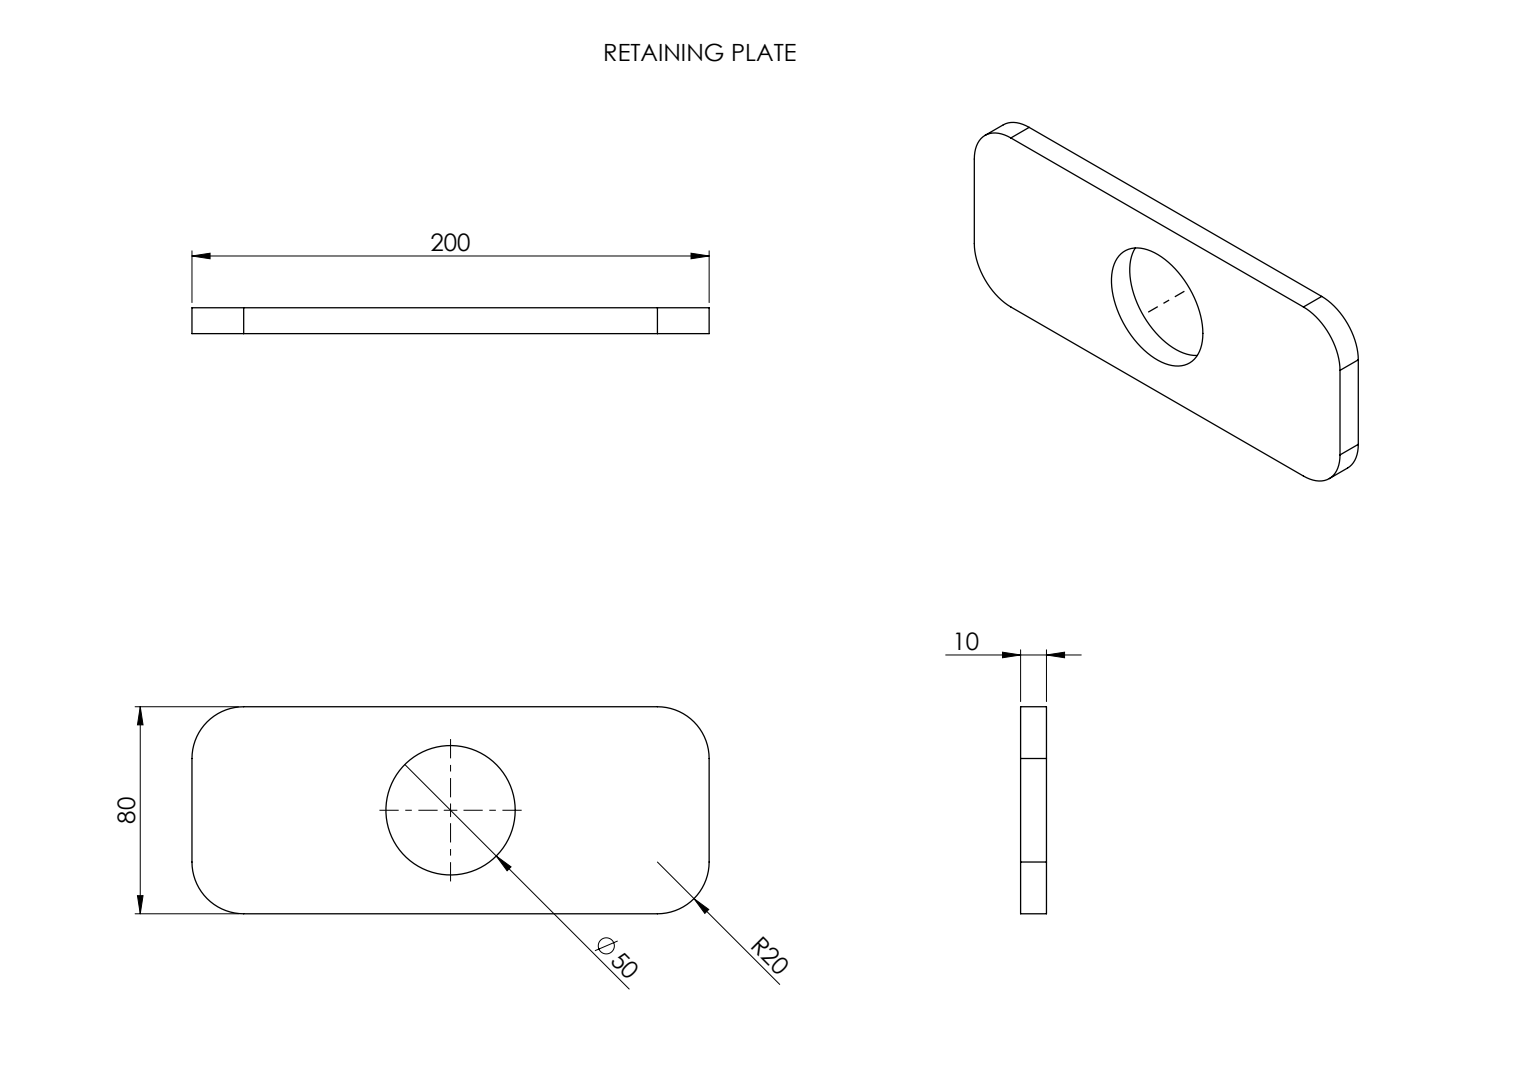
ISO-10303-21;
HEADER;
FILE_DESCRIPTION (('STEP AP203'),
    '1' );
FILE_NAME ('retaining plate.step',
    '2026-09-28T05:57:06',
    ( '' ),
    ( '' ),
    'SwSTEP 2.0',
    'SolidWorks 2026',
    '' );
FILE_SCHEMA (( 'AUTOMOTIVE_DESIGN' ));
ENDSEC;

DATA;
#122=DIRECTION ( 'NONE',  ( -1.000000000000000000, 0.000000000000000000, 0.000000000000000000 ) ) ;
#133=AXIS2_PLACEMENT_3D ( 'NONE', #27318, #14555, #30777 ) ;
#134=VERTEX_POINT ( 'NONE', #10468 ) ;
#200=CYLINDRICAL_SURFACE ( 'NONE', #38257, 25.00000000000000000 ) ;
#235=CARTESIAN_POINT ( 'NONE',  ( 0.000000000000000000, 0.000000000000000000, -170.0000000000000000 ) ) ;
#587=VERTEX_POINT ( 'NONE', #37224 ) ;
#645=EDGE_CURVE ( 'NONE', #15029, #36871, #9699, .T. ) ;
#867=CARTESIAN_POINT ( 'NONE',  ( 80.00000000000002842, 19.99999999999999289, -160.0000000000000000 ) ) ;
#917=DIRECTION ( 'NONE',  ( 0.000000000000000000, 0.000000000000000000, -1.000000000000000000 ) ) ;
#1054=VERTEX_POINT ( 'NONE', #16453 ) ;
#1121=CIRCLE ( 'NONE', #7312, 20.00000000000000355 ) ;
#1204=MANIFOLD_SOLID_BREP ( 'Fillet1', #25326 ) ;
#1238=VECTOR ( 'NONE', #42446, 1000.000000000000000 ) ;
#1422=DIRECTION ( 'NONE',  ( -0.000000000000000000, -0.000000000000000000, 1.000000000000000000 ) ) ;
#1650=VERTEX_POINT ( 'NONE', #15142 ) ;
#1704=ORIENTED_EDGE ( 'NONE', *, *, #24624, .F. ) ;
#1835=EDGE_CURVE ( 'NONE', #1650, #37987, #25230, .T. ) ;
#2068=EDGE_LOOP ( 'NONE', ( #40227, #42312 ) ) ;
#2131=ORIENTED_EDGE ( 'NONE', *, *, #9361, .F. ) ;
#2180=LINE ( 'NONE', #18985, #13807 ) ;
#2200=VECTOR ( 'NONE', #3034, 1000.000000000000000 ) ;
#2225=FACE_OUTER_BOUND ( 'NONE', #37868, .T. ) ;
#2336=DIRECTION ( 'NONE',  ( -1.000000000000000000, 0.000000000000000000, 0.000000000000000000 ) ) ;
#2490=AXIS2_PLACEMENT_3D ( 'NONE', #26366, #42534, #23345 ) ;
#2545=DIRECTION ( 'NONE',  ( 0.000000000000000000, 0.000000000000000000, -1.000000000000000000 ) ) ;
#2726=AXIS2_PLACEMENT_3D ( 'NONE', #867, #39910, #20909 ) ;
#2917=DIRECTION ( 'NONE',  ( 0.000000000000000000, 0.000000000000000000, -1.000000000000000000 ) ) ;
#3034=DIRECTION ( 'NONE',  ( -0.000000000000000000, -0.000000000000000000, 1.000000000000000000 ) ) ;
#3160=DIRECTION ( 'NONE',  ( -0.000000000000000000, -0.000000000000000000, -1.000000000000000000 ) ) ;
#3228=VERTEX_POINT ( 'NONE', #30090 ) ;
#3281=PRODUCT_DEFINITION ( 'UNKNOWN', '', #22864, #26130 ) ;
#3291=AXIS2_PLACEMENT_3D ( 'NONE', #10282, #23469, #36616 ) ;
#3398=VECTOR ( 'NONE', #23149, 1000.000000000000000 ) ;
#3399=FACE_BOUND ( 'NONE', #39258, .T. ) ;
#3599=DIRECTION ( 'NONE',  ( -1.000000000000000000, 0.000000000000000000, 0.000000000000000000 ) ) ;
#3726=DIRECTION ( 'NONE',  ( -1.000000000000000000, -1.734723475976806848E-16, 0.000000000000000000 ) ) ;
#3807=CIRCLE ( 'NONE', #15519, 20.00000000000000355 ) ;
#3812=ORIENTED_EDGE ( 'NONE', *, *, #16436, .F. ) ;
#3857=ORIENTED_EDGE ( 'NONE', *, *, #28973, .F. ) ;
#3901=VECTOR ( 'NONE', #38849, 1000.000000000000000 ) ;
#4172=VERTEX_POINT ( 'NONE', #30883 ) ;
#4780=CARTESIAN_POINT ( 'NONE',  ( -99.99999999999994316, 19.99999999999998934, -160.0000000000000000 ) ) ;
#4830=DIRECTION ( 'NONE',  ( 0.000000000000000000, 0.000000000000000000, -1.000000000000000000 ) ) ;
#4866=DIRECTION ( 'NONE',  ( 0.000000000000000000, 0.000000000000000000, -1.000000000000000000 ) ) ;
#4920=DIRECTION ( 'NONE',  ( 0.000000000000000000, 0.000000000000000000, -1.000000000000000000 ) ) ;
#5144=ORIENTED_EDGE ( 'NONE', *, *, #23603, .F. ) ;
#5298=( NAMED_UNIT ( * ) SI_UNIT ( $, .STERADIAN. ) SOLID_ANGLE_UNIT ( ) );
#5409=CARTESIAN_POINT ( 'NONE',  ( -99.99999999999994316, 39.99999999999999289, -160.0000000000000000 ) ) ;
#5497=ORIENTED_EDGE ( 'NONE', *, *, #20467, .F. ) ;
#5582=AXIS2_PLACEMENT_3D ( 'NONE', #18873, #12589, #31631 ) ;
#5609=EDGE_LOOP ( 'NONE', ( #14936, #24531, #13344, #38796 ) ) ;
#5623=EDGE_LOOP ( 'NONE', ( #1704, #31810, #14532, #33862 ) ) ;
#6178=VECTOR ( 'NONE', #4830, 1000.000000000000000 ) ;
#6245=ORIENTED_EDGE ( 'NONE', *, *, #24624, .T. ) ;
#6332=VECTOR ( 'NONE', #39526, 1000.000000000000000 ) ;
#6411=CARTESIAN_POINT ( 'NONE',  ( 100.0000000000000284, -40.00000000000001421, -160.0000000000000000 ) ) ;
#6686=LINE ( 'NONE', #36256, #2200 ) ;
#6890=ORIENTED_EDGE ( 'NONE', *, *, #8772, .T. ) ;
#6921=ORIENTED_EDGE ( 'NONE', *, *, #32093, .F. ) ;
#6955=FACE_OUTER_BOUND ( 'NONE', #37730, .T. ) ;
#7119=DIRECTION ( 'NONE',  ( -0.000000000000000000, -0.000000000000000000, -1.000000000000000000 ) ) ;
#7120=DIRECTION ( 'NONE',  ( -0.000000000000000000, -0.000000000000000000, 1.000000000000000000 ) ) ;
#7230=ADVANCED_FACE ( 'NONE', ( #39848 ), #16746, .F. ) ;
#7298=DIRECTION ( 'NONE',  ( 0.000000000000000000, 0.000000000000000000, 1.000000000000000000 ) ) ;
#7312=AXIS2_PLACEMENT_3D ( 'NONE', #35263, #14357, #27554 ) ;
#7469=ADVANCED_FACE ( 'NONE', ( #32970, #3399 ), #16534, .F. ) ;
#7703=APPLICATION_CONTEXT ( 'configuration controlled 3d designs of mechanical parts and assemblies' ) ;
#7767=CARTESIAN_POINT ( 'NONE',  ( -79.99999999999994316, -20.00000000000000711, -160.0000000000000000 ) ) ;
#7802=FACE_OUTER_BOUND ( 'NONE', #41194, .T. ) ;
#7902=DIRECTION ( 'NONE',  ( 0.000000000000000000, 0.000000000000000000, 1.000000000000000000 ) ) ;
#8162=CARTESIAN_POINT ( 'NONE',  ( 0.000000000000000000, 0.000000000000000000, -170.0000000000000000 ) ) ;
#8437=EDGE_CURVE ( 'NONE', #3228, #21146, #34411, .T. ) ;
#8559=LINE ( 'NONE', #24974, #41909 ) ;
#8607=DIRECTION ( 'NONE',  ( 1.000000000000000000, -3.469446951953614805E-17, 0.000000000000000000 ) ) ;
#8772=EDGE_CURVE ( 'NONE', #21146, #4172, #25761, .T. ) ;
#8901=EDGE_CURVE ( 'NONE', #1054, #27758, #21322, .T. ) ;
#8918=CIRCLE ( 'NONE', #16462, 25.00000000000000000 ) ;
#9272=MECHANICAL_CONTEXT ( 'NONE', #7703, 'mechanical' ) ;
#9361=EDGE_CURVE ( 'NONE', #36871, #15029, #8918, .T. ) ;
#9371=ORIENTED_EDGE ( 'NONE', *, *, #8772, .F. ) ;
#9378=SHAPE_REPRESENTATION_RELATIONSHIP ( 'NONE' , 'NONE' ,  #10057, #19190 ) ;
#9407=VERTEX_POINT ( 'NONE', #26337 ) ;
#9447=LINE ( 'NONE', #31923, #1238 ) ;
#9492=ORIENTED_EDGE ( 'NONE', *, *, #21192, .T. ) ;
#9586=EDGE_LOOP ( 'NONE', ( #5144, #34825, #5497, #32629 ) ) ;
#9592=ADVANCED_FACE ( 'NONE', ( #26124 ), #22894, .T. ) ;
#9637=CYLINDRICAL_SURFACE ( 'NONE', #9748, 20.00000000000000355 ) ;
#9699=CIRCLE ( 'NONE', #5582, 25.00000000000000000 ) ;
#9748=AXIS2_PLACEMENT_3D ( 'NONE', #35973, #19551, #3599 ) ;
#9837=EDGE_CURVE ( 'NONE', #35669, #36871, #20483, .T. ) ;
#9969=DIRECTION ( 'NONE',  ( 0.000000000000000000, 0.000000000000000000, -1.000000000000000000 ) ) ;
#10057=SHAPE_REPRESENTATION ( 'retaining plate', ( #39998 ), #28334 ) ;
#10182=CARTESIAN_POINT ( 'NONE',  ( -99.99999999999994316, -40.00000000000000711, -170.0000000000000000 ) ) ;
#10282=CARTESIAN_POINT ( 'NONE',  ( -99.99999999999994316, -40.00000000000000711, -160.0000000000000000 ) ) ;
#10468=CARTESIAN_POINT ( 'NONE',  ( 25.00000000000000000, 3.061616997868383043E-15, -160.0000000000000000 ) ) ;
#11095=CYLINDRICAL_SURFACE ( 'NONE', #30680, 20.00000000000000355 ) ;
#11112=DIRECTION ( 'NONE',  ( 0.000000000000000000, 0.000000000000000000, 1.000000000000000000 ) ) ;
#11120=LINE ( 'NONE', #41104, #22218 ) ;
#11183=DIRECTION ( 'NONE',  ( -0.000000000000000000, -0.000000000000000000, 1.000000000000000000 ) ) ;
#11249=CARTESIAN_POINT ( 'NONE',  ( 80.00000000000002842, 39.99999999999999289, -160.0000000000000000 ) ) ;
#11303=ORIENTED_EDGE ( 'NONE', *, *, #29515, .F. ) ;
#11345=DIRECTION ( 'NONE',  ( 0.000000000000000000, 0.000000000000000000, -1.000000000000000000 ) ) ;
#11759=ORIENTED_EDGE ( 'NONE', *, *, #37514, .F. ) ;
#12340=ADVANCED_FACE ( 'NONE', ( #15920 ), #200, .F. ) ;
#12589=DIRECTION ( 'NONE',  ( 0.000000000000000000, 0.000000000000000000, 1.000000000000000000 ) ) ;
#12653=ORIENTED_EDGE ( 'NONE', *, *, #16256, .T. ) ;
#13051=ORIENTED_EDGE ( 'NONE', *, *, #8437, .T. ) ;
#13321=DIRECTION ( 'NONE',  ( -0.000000000000000000, -0.000000000000000000, -1.000000000000000000 ) ) ;
#13344=ORIENTED_EDGE ( 'NONE', *, *, #32270, .F. ) ;
#13404=CARTESIAN_POINT ( 'NONE',  ( 100.0000000000000284, -40.00000000000001421, -160.0000000000000000 ) ) ;
#13464=ORIENTED_EDGE ( 'NONE', *, *, #9837, .F. ) ;
#13490=CARTESIAN_POINT ( 'NONE',  ( 100.0000000000000142, 19.99999999999999645, -170.0000000000000000 ) ) ;
#13514=ADVANCED_FACE ( 'NONE', ( #28385 ), #11095, .T. ) ;
#13644=AXIS2_PLACEMENT_3D ( 'NONE', #13404, #3726, #33301 ) ;
#13744=CIRCLE ( 'NONE', #37172, 25.00000000000000000 ) ;
#13807=VECTOR ( 'NONE', #32172, 1000.000000000000000 ) ;
#14070=EDGE_LOOP ( 'NONE', ( #18613, #15321, #9371, #33335, #11303, #26518, #40941, #34241 ) ) ;
#14116=CYLINDRICAL_SURFACE ( 'NONE', #133, 25.00000000000000000 ) ;
#14322=EDGE_CURVE ( 'NONE', #27758, #41802, #26584, .T. ) ;
#14357=DIRECTION ( 'NONE',  ( 0.000000000000000000, 0.000000000000000000, -1.000000000000000000 ) ) ;
#14532=ORIENTED_EDGE ( 'NONE', *, *, #9837, .T. ) ;
#14555=DIRECTION ( 'NONE',  ( -0.000000000000000000, -0.000000000000000000, -1.000000000000000000 ) ) ;
#14810=VECTOR ( 'NONE', #3160, 1000.000000000000000 ) ;
#14936=ORIENTED_EDGE ( 'NONE', *, *, #1835, .F. ) ;
#15029=VERTEX_POINT ( 'NONE', #23301 ) ;
#15052=CARTESIAN_POINT ( 'NONE',  ( -99.99999999999994316, -20.00000000000000355, -160.0000000000000000 ) ) ;
#15142=CARTESIAN_POINT ( 'NONE',  ( -79.99999999999992895, 39.99999999999999289, -160.0000000000000000 ) ) ;
#15265=AXIS2_PLACEMENT_3D ( 'NONE', #30995, #1422, #17367 ) ;
#15321=ORIENTED_EDGE ( 'NONE', *, *, #22014, .T. ) ;
#15352=DIRECTION ( 'NONE',  ( 1.000000000000000000, -1.734723475976807094E-16, 0.000000000000000000 ) ) ;
#15519=AXIS2_PLACEMENT_3D ( 'NONE', #7767, #7120, #17237 ) ;
#15595=CARTESIAN_POINT ( 'NONE',  ( 80.00000000000002842, 19.99999999999999289, -160.0000000000000000 ) ) ;
#15920=FACE_OUTER_BOUND ( 'NONE', #5623, .T. ) ;
#16047=DIRECTION ( 'NONE',  ( -1.000000000000000000, 0.000000000000000000, 0.000000000000000000 ) ) ;
#16132=DIRECTION ( 'NONE',  ( 1.000000000000000000, 0.000000000000000000, 0.000000000000000000 ) ) ;
#16134=ORIENTED_EDGE ( 'NONE', *, *, #27689, .F. ) ;
#16256=EDGE_CURVE ( 'NONE', #4172, #35088, #21152, .T. ) ;
#16436=EDGE_CURVE ( 'NONE', #28405, #1650, #34982, .T. ) ;
#16453=CARTESIAN_POINT ( 'NONE',  ( 80.00000000000002842, 39.99999999999999289, -170.0000000000000000 ) ) ;
#16462=AXIS2_PLACEMENT_3D ( 'NONE', #235, #35638, #19843 ) ;
#16504=CARTESIAN_POINT ( 'NONE',  ( 25.00000000000000000, 3.061616997868383043E-15, -160.0000000000000000 ) ) ;
#16534=PLANE ( 'NONE',  #32965 ) ;
#16746=PLANE ( 'NONE',  #3291 ) ;
#16764=CARTESIAN_POINT ( 'NONE',  ( -25.00000000000000000, 0.000000000000000000, -160.0000000000000000 ) ) ;
#17214=ORIENTED_EDGE ( 'NONE', *, *, #28094, .T. ) ;
#17237=DIRECTION ( 'NONE',  ( -1.000000000000000000, 0.000000000000000000, 0.000000000000000000 ) ) ;
#17244=CARTESIAN_POINT ( 'NONE',  ( 79.99999999999998579, -40.00000000000001421, -160.0000000000000000 ) ) ;
#17307=PRODUCT_DEFINITION_SHAPE ( 'NONE', 'NONE',  #3281 ) ;
#17367=DIRECTION ( 'NONE',  ( -1.000000000000000000, 8.673617379884033500E-16, 0.000000000000000000 ) ) ;
#17762=CARTESIAN_POINT ( 'NONE',  ( -79.99999999999994316, -40.00000000000000711, -160.0000000000000000 ) ) ;
#17912=EDGE_LOOP ( 'NONE', ( #35232, #35494, #28919, #22817 ) ) ;
#18014=ADVANCED_FACE ( 'NONE', ( #2225 ), #25937, .F. ) ;
#18558=AXIS2_PLACEMENT_3D ( 'NONE', #39539, #9969, #40803 ) ;
#18559=DIRECTION ( 'NONE',  ( -1.000000000000000000, -0.000000000000000000, -0.000000000000000000 ) ) ;
#18613=ORIENTED_EDGE ( 'NONE', *, *, #41740, .F. ) ;
#18630=AXIS2_PLACEMENT_3D ( 'NONE', #22383, #2545, #2336 ) ;
#18665=ORIENTED_EDGE ( 'NONE', *, *, #37514, .T. ) ;
#18724=VECTOR ( 'NONE', #4866, 1000.000000000000000 ) ;
#18772=EDGE_LOOP ( 'NONE', ( #6890, #12653, #3857, #13051 ) ) ;
#18873=CARTESIAN_POINT ( 'NONE',  ( 0.000000000000000000, 0.000000000000000000, -170.0000000000000000 ) ) ;
#18985=CARTESIAN_POINT ( 'NONE',  ( 100.0000000000000284, -40.00000000000001421, -170.0000000000000000 ) ) ;
#19044=EDGE_CURVE ( 'NONE', #134, #35669, #40833, .T. ) ;
#19190=ADVANCED_BREP_SHAPE_REPRESENTATION ( '', ( #1204, #39998 ), #28334 ) ;
#19296=CARTESIAN_POINT ( 'NONE',  ( -79.99999999999994316, -20.00000000000000711, -170.0000000000000000 ) ) ;
#19355=ORIENTED_EDGE ( 'NONE', *, *, #16256, .F. ) ;
#19531=VERTEX_POINT ( 'NONE', #31171 ) ;
#19551=DIRECTION ( 'NONE',  ( 0.000000000000000000, 0.000000000000000000, -1.000000000000000000 ) ) ;
#19843=DIRECTION ( 'NONE',  ( 1.000000000000000000, 0.000000000000000000, 0.000000000000000000 ) ) ;
#20056=CARTESIAN_POINT ( 'NONE',  ( -25.00000000000000000, 0.000000000000000000, -160.0000000000000000 ) ) ;
#20094=VECTOR ( 'NONE', #23232, 1000.000000000000000 ) ;
#20100=APPLICATION_CONTEXT ( 'configuration controlled 3d designs of mechanical parts and assemblies' ) ;
#20112=PLANE ( 'NONE',  #13644 ) ;
#20145=AXIS2_PLACEMENT_3D ( 'NONE', #28763, #15352, #28967 ) ;
#20467=EDGE_CURVE ( 'NONE', #21146, #40566, #38983, .T. ) ;
#20483=LINE ( 'NONE', #20056, #33048 ) ;
#20586=CIRCLE ( 'NONE', #41943, 20.00000000000000355 ) ;
#20890=ADVANCED_FACE ( 'NONE', ( #7802 ), #24209, .F. ) ;
#20909=DIRECTION ( 'NONE',  ( -1.000000000000000000, 0.000000000000000000, 0.000000000000000000 ) ) ;
#20950=CARTESIAN_POINT ( 'NONE',  ( -99.99999999999994316, 39.99999999999999289, -160.0000000000000000 ) ) ;
#21146=VERTEX_POINT ( 'NONE', #38213 ) ;
#21152=LINE ( 'NONE', #25060, #40780 ) ;
#21192=EDGE_CURVE ( 'NONE', #1054, #19531, #28520, .T. ) ;
#21322=CIRCLE ( 'NONE', #18558, 20.00000000000000355 ) ;
#21369=DIRECTION ( 'NONE',  ( -0.000000000000000000, -0.000000000000000000, 1.000000000000000000 ) ) ;
#21474=LINE ( 'NONE', #38513, #18724 ) ;
#21599=DIRECTION ( 'NONE',  ( 0.000000000000000000, -0.000000000000000000, -1.000000000000000000 ) ) ;
#21848=PRODUCT ( 'retaining plate', 'retaining plate', '', ( #9272 ) ) ;
#21900=VECTOR ( 'NONE', #11183, 1000.000000000000000 ) ;
#22014=EDGE_CURVE ( 'NONE', #9407, #4172, #1121, .T. ) ;
#22076=ORIENTED_EDGE ( 'NONE', *, *, #32093, .T. ) ;
#22218=VECTOR ( 'NONE', #24752, 1000.000000000000000 ) ;
#22383=CARTESIAN_POINT ( 'NONE',  ( -79.99999999999992895, 19.99999999999998934, -160.0000000000000000 ) ) ;
#22593=CYLINDRICAL_SURFACE ( 'NONE', #18630, 20.00000000000000355 ) ;
#22763=ORIENTED_EDGE ( 'NONE', *, *, #22014, .F. ) ;
#22817=ORIENTED_EDGE ( 'NONE', *, *, #28094, .F. ) ;
#22864=PRODUCT_DEFINITION_FORMATION_WITH_SPECIFIED_SOURCE ( 'ANY', '', #21848, .NOT_KNOWN. ) ;
#22894=CYLINDRICAL_SURFACE ( 'NONE', #2726, 20.00000000000000355 ) ;
#22917=VECTOR ( 'NONE', #18559, 1000.000000000000000 ) ;
#22926=ORIENTED_EDGE ( 'NONE', *, *, #31024, .T. ) ;
#23062=CARTESIAN_POINT ( 'NONE',  ( 0.000000000000000000, 0.000000000000000000, -160.0000000000000000 ) ) ;
#23149=DIRECTION ( 'NONE',  ( 1.000000000000000000, -3.469446951953614805E-17, 0.000000000000000000 ) ) ;
#23232=DIRECTION ( 'NONE',  ( -1.734723475976806848E-16, 1.000000000000000000, 0.000000000000000000 ) ) ;
#23301=CARTESIAN_POINT ( 'NONE',  ( 25.00000000000000000, 3.061616997868383043E-15, -170.0000000000000000 ) ) ;
#23345=DIRECTION ( 'NONE',  ( -1.000000000000000000, 0.000000000000000000, 0.000000000000000000 ) ) ;
#23452=AXIS2_PLACEMENT_3D ( 'NONE', #8162, #4920, #41145 ) ;
#23469=DIRECTION ( 'NONE',  ( 3.469446951953614805E-17, 1.000000000000000000, -0.000000000000000000 ) ) ;
#23603=EDGE_CURVE ( 'NONE', #587, #3228, #3807, .T. ) ;
#24209=PLANE ( 'NONE',  #27991 ) ;
#24312=CARTESIAN_POINT ( 'NONE',  ( -99.99999999999994316, -20.00000000000000355, -170.0000000000000000 ) ) ;
#24380=LINE ( 'NONE', #15052, #21900 ) ;
#24531=ORIENTED_EDGE ( 'NONE', *, *, #27009, .F. ) ;
#24572=PLANE ( 'NONE',  #23452 ) ;
#24624=EDGE_CURVE ( 'NONE', #134, #15029, #39192, .T. ) ;
#24641=DIRECTION ( 'NONE',  ( 0.000000000000000000, -1.000000000000000000, 0.000000000000000000 ) ) ;
#24743=CARTESIAN_POINT ( 'NONE',  ( 0.000000000000000000, 0.000000000000000000, 0.000000000000000000 ) ) ;
#24752=DIRECTION ( 'NONE',  ( -1.734723475976807094E-16, -1.000000000000000000, -0.000000000000000000 ) ) ;
#24940=DIRECTION ( 'NONE',  ( -1.000000000000000000, 0.000000000000000000, 0.000000000000000000 ) ) ;
#24974=CARTESIAN_POINT ( 'NONE',  ( 100.0000000000000284, -20.00000000000001066, -160.0000000000000000 ) ) ;
#25060=CARTESIAN_POINT ( 'NONE',  ( 80.00000000000004263, -40.00000000000001421, -160.0000000000000000 ) ) ;
#25111=ORIENTED_EDGE ( 'NONE', *, *, #29515, .T. ) ;
#25197=CARTESIAN_POINT ( 'NONE',  ( -25.00000000000000000, 0.000000000000000000, -170.0000000000000000 ) ) ;
#25230=CIRCLE ( 'NONE', #2490, 20.00000000000000355 ) ;
#25326=CLOSED_SHELL ( 'NONE', ( #28078, #7469, #41143, #32960, #20890, #18014, #7230, #12340, #27771, #9592, #13514, #41382 ) ) ;
#25638=ORIENTED_EDGE ( 'NONE', *, *, #1835, .T. ) ;
#25761=LINE ( 'NONE', #10182, #3398 ) ;
#25937=PLANE ( 'NONE',  #20145 ) ;
#26124=FACE_OUTER_BOUND ( 'NONE', #17912, .T. ) ;
#26130=DESIGN_CONTEXT ( 'detailed design', #20100, 'design' ) ;
#26337=CARTESIAN_POINT ( 'NONE',  ( 100.0000000000000284, -20.00000000000001066, -170.0000000000000000 ) ) ;
#26366=CARTESIAN_POINT ( 'NONE',  ( -79.99999999999992895, 19.99999999999998934, -160.0000000000000000 ) ) ;
#26518=ORIENTED_EDGE ( 'NONE', *, *, #32270, .T. ) ;
#26584=LINE ( 'NONE', #29402, #6332 ) ;
#26744=VERTEX_POINT ( 'NONE', #31979 ) ;
#26770=CIRCLE ( 'NONE', #33680, 20.00000000000000355 ) ;
#27009=EDGE_CURVE ( 'NONE', #19531, #1650, #6686, .T. ) ;
#27318=CARTESIAN_POINT ( 'NONE',  ( 0.000000000000000000, 0.000000000000000000, -160.0000000000000000 ) ) ;
#27323=CARTESIAN_POINT ( 'NONE',  ( 0.000000000000000000, 0.000000000000000000, -160.0000000000000000 ) ) ;
#27532=FACE_OUTER_BOUND ( 'NONE', #37603, .T. ) ;
#27554=DIRECTION ( 'NONE',  ( -1.000000000000000000, 0.000000000000000000, 0.000000000000000000 ) ) ;
#27584=FACE_OUTER_BOUND ( 'NONE', #14070, .T. ) ;
#27681=ORIENTED_EDGE ( 'NONE', *, *, #23603, .T. ) ;
#27689=EDGE_CURVE ( 'NONE', #26744, #41802, #39830, .T. ) ;
#27758=VERTEX_POINT ( 'NONE', #13490 ) ;
#27771=ADVANCED_FACE ( 'NONE', ( #39411 ), #9637, .T. ) ;
#27968=EDGE_CURVE ( 'NONE', #35088, #26744, #33902, .T. ) ;
#27991=AXIS2_PLACEMENT_3D ( 'NONE', #20950, #24641, #21599 ) ;
#28078=ADVANCED_FACE ( 'NONE', ( #27532 ), #14116, .F. ) ;
#28094=EDGE_CURVE ( 'NONE', #28405, #1054, #21474, .T. ) ;
#28165=ORIENTED_EDGE ( 'NONE', *, *, #31256, .F. ) ;
#28334=( GEOMETRIC_REPRESENTATION_CONTEXT ( 3 ) GLOBAL_UNCERTAINTY_ASSIGNED_CONTEXT ( ( #39784 ) ) GLOBAL_UNIT_ASSIGNED_CONTEXT ( ( #40886, #38945, #5298 ) ) REPRESENTATION_CONTEXT ( 'NONE', 'WORKASPACE' ) );
#28385=FACE_OUTER_BOUND ( 'NONE', #9586, .T. ) ;
#28405=VERTEX_POINT ( 'NONE', #11249 ) ;
#28470=CARTESIAN_POINT ( 'NONE',  ( -99.99999999999994316, -40.00000000000000711, -160.0000000000000000 ) ) ;
#28520=LINE ( 'NONE', #35201, #3901 ) ;
#28561=ORIENTED_EDGE ( 'NONE', *, *, #33231, .T. ) ;
#28763=CARTESIAN_POINT ( 'NONE',  ( -99.99999999999994316, -40.00000000000000711, -160.0000000000000000 ) ) ;
#28797=DIRECTION ( 'NONE',  ( -1.000000000000000000, 0.000000000000000000, 0.000000000000000000 ) ) ;
#28820=ORIENTED_EDGE ( 'NONE', *, *, #34065, .T. ) ;
#28919=ORIENTED_EDGE ( 'NONE', *, *, #8901, .F. ) ;
#28967=DIRECTION ( 'NONE',  ( 1.734723475976807094E-16, 1.000000000000000000, 0.000000000000000000 ) ) ;
#28973=EDGE_CURVE ( 'NONE', #3228, #35088, #38374, .T. ) ;
#29402=CARTESIAN_POINT ( 'NONE',  ( 100.0000000000000142, 19.99999999999999645, -160.0000000000000000 ) ) ;
#29515=EDGE_CURVE ( 'NONE', #34935, #40566, #11120, .T. ) ;
#29658=ORIENTED_EDGE ( 'NONE', *, *, #41740, .T. ) ;
#29732=CARTESIAN_POINT ( 'NONE',  ( 0.000000000000000000, 0.000000000000000000, -160.0000000000000000 ) ) ;
#30090=CARTESIAN_POINT ( 'NONE',  ( -79.99999999999995737, -40.00000000000000711, -160.0000000000000000 ) ) ;
#30093=ORIENTED_EDGE ( 'NONE', *, *, #27968, .F. ) ;
#30489=LINE ( 'NONE', #4780, #39176 ) ;
#30680=AXIS2_PLACEMENT_3D ( 'NONE', #31198, #34434, #24940 ) ;
#30777=DIRECTION ( 'NONE',  ( -1.000000000000000000, 0.000000000000000000, 0.000000000000000000 ) ) ;
#30883=CARTESIAN_POINT ( 'NONE',  ( 79.99999999999998579, -40.00000000000001421, -170.0000000000000000 ) ) ;
#30995=CARTESIAN_POINT ( 'NONE',  ( 80.00000000000002842, -20.00000000000001421, -160.0000000000000000 ) ) ;
#31024=EDGE_CURVE ( 'NONE', #40566, #587, #24380, .T. ) ;
#31171=CARTESIAN_POINT ( 'NONE',  ( -79.99999999999992895, 39.99999999999999289, -170.0000000000000000 ) ) ;
#31198=CARTESIAN_POINT ( 'NONE',  ( -79.99999999999994316, -20.00000000000000711, -160.0000000000000000 ) ) ;
#31256=EDGE_CURVE ( 'NONE', #37987, #587, #9447, .T. ) ;
#31631=DIRECTION ( 'NONE',  ( 1.000000000000000000, 0.000000000000000000, 0.000000000000000000 ) ) ;
#31810=ORIENTED_EDGE ( 'NONE', *, *, #19044, .T. ) ;
#31906=FACE_OUTER_BOUND ( 'NONE', #5609, .T. ) ;
#31923=CARTESIAN_POINT ( 'NONE',  ( -99.99999999999994316, -40.00000000000000711, -160.0000000000000000 ) ) ;
#31979=CARTESIAN_POINT ( 'NONE',  ( 100.0000000000000284, -20.00000000000001066, -160.0000000000000000 ) ) ;
#32093=EDGE_CURVE ( 'NONE', #26744, #9407, #8559, .T. ) ;
#32172=DIRECTION ( 'NONE',  ( -1.734723475976806848E-16, 1.000000000000000000, 0.000000000000000000 ) ) ;
#32270=EDGE_CURVE ( 'NONE', #34935, #19531, #26770, .T. ) ;
#32629=ORIENTED_EDGE ( 'NONE', *, *, #8437, .F. ) ;
#32960=ADVANCED_FACE ( 'NONE', ( #6955 ), #20112, .F. ) ;
#32965=AXIS2_PLACEMENT_3D ( 'NONE', #29732, #11345, #40903 ) ;
#32970=FACE_OUTER_BOUND ( 'NONE', #40050, .T. ) ;
#33048=VECTOR ( 'NONE', #7119, 1000.000000000000000 ) ;
#33145=ORIENTED_EDGE ( 'NONE', *, *, #19044, .F. ) ;
#33151=ORIENTED_EDGE ( 'NONE', *, *, #27689, .T. ) ;
#33231=EDGE_CURVE ( 'NONE', #37987, #34935, #30489, .T. ) ;
#33301=DIRECTION ( 'NONE',  ( 1.734723475976806848E-16, -1.000000000000000000, 0.000000000000000000 ) ) ;
#33335=ORIENTED_EDGE ( 'NONE', *, *, #20467, .T. ) ;
#33680=AXIS2_PLACEMENT_3D ( 'NONE', #39793, #39373, #122 ) ;
#33862=ORIENTED_EDGE ( 'NONE', *, *, #645, .F. ) ;
#33902=CIRCLE ( 'NONE', #15265, 20.00000000000000355 ) ;
#33968=ORIENTED_EDGE ( 'NONE', *, *, #14322, .T. ) ;
#34065=EDGE_CURVE ( 'NONE', #41802, #28405, #20586, .T. ) ;
#34130=ORIENTED_EDGE ( 'NONE', *, *, #27009, .T. ) ;
#34241=ORIENTED_EDGE ( 'NONE', *, *, #8901, .T. ) ;
#34411=LINE ( 'NONE', #17762, #6178 ) ;
#34434=DIRECTION ( 'NONE',  ( 0.000000000000000000, 0.000000000000000000, -1.000000000000000000 ) ) ;
#34825=ORIENTED_EDGE ( 'NONE', *, *, #31024, .F. ) ;
#34935=VERTEX_POINT ( 'NONE', #35853 ) ;
#34982=LINE ( 'NONE', #5409, #22917 ) ;
#35088=VERTEX_POINT ( 'NONE', #17244 ) ;
#35201=CARTESIAN_POINT ( 'NONE',  ( -99.99999999999994316, 39.99999999999999289, -170.0000000000000000 ) ) ;
#35232=ORIENTED_EDGE ( 'NONE', *, *, #34065, .F. ) ;
#35263=CARTESIAN_POINT ( 'NONE',  ( 80.00000000000002842, -20.00000000000001421, -170.0000000000000000 ) ) ;
#35360=AXIS2_PLACEMENT_3D ( 'NONE', #36855, #7298, #16132 ) ;
#35494=ORIENTED_EDGE ( 'NONE', *, *, #14322, .F. ) ;
#35638=DIRECTION ( 'NONE',  ( 0.000000000000000000, 0.000000000000000000, 1.000000000000000000 ) ) ;
#35669=VERTEX_POINT ( 'NONE', #16764 ) ;
#35853=CARTESIAN_POINT ( 'NONE',  ( -99.99999999999994316, 19.99999999999998934, -170.0000000000000000 ) ) ;
#35973=CARTESIAN_POINT ( 'NONE',  ( 80.00000000000002842, -20.00000000000001421, -160.0000000000000000 ) ) ;
#36256=CARTESIAN_POINT ( 'NONE',  ( -79.99999999999992895, 39.99999999999999289, -160.0000000000000000 ) ) ;
#36596=CARTESIAN_POINT ( 'NONE',  ( -99.99999999999994316, 19.99999999999998934, -160.0000000000000000 ) ) ;
#36616=DIRECTION ( 'NONE',  ( -1.000000000000000000, 3.469446951953614805E-17, 0.000000000000000000 ) ) ;
#36819=ORIENTED_EDGE ( 'NONE', *, *, #27968, .T. ) ;
#36855=CARTESIAN_POINT ( 'NONE',  ( 0.000000000000000000, 0.000000000000000000, -160.0000000000000000 ) ) ;
#36869=CARTESIAN_POINT ( 'NONE',  ( 100.0000000000000142, 19.99999999999999645, -160.0000000000000000 ) ) ;
#36871=VERTEX_POINT ( 'NONE', #25197 ) ;
#37172=AXIS2_PLACEMENT_3D ( 'NONE', #27323, #7902, #37674 ) ;
#37224=CARTESIAN_POINT ( 'NONE',  ( -99.99999999999994316, -20.00000000000000355, -160.0000000000000000 ) ) ;
#37514=EDGE_CURVE ( 'NONE', #35669, #134, #13744, .T. ) ;
#37603=EDGE_LOOP ( 'NONE', ( #18665, #6245, #2131, #13464 ) ) ;
#37620=AXIS2_PLACEMENT_3D ( 'NONE', #19296, #2917, #16047 ) ;
#37674=DIRECTION ( 'NONE',  ( 1.000000000000000000, 0.000000000000000000, 0.000000000000000000 ) ) ;
#37730=EDGE_LOOP ( 'NONE', ( #16134, #22076, #29658, #33968 ) ) ;
#37868=EDGE_LOOP ( 'NONE', ( #25111, #22926, #28165, #28561 ) ) ;
#37889=DIRECTION ( 'NONE',  ( 1.000000000000000000, 0.000000000000000000, 0.000000000000000000 ) ) ;
#37987=VERTEX_POINT ( 'NONE', #36596 ) ;
#38213=CARTESIAN_POINT ( 'NONE',  ( -79.99999999999995737, -40.00000000000000711, -170.0000000000000000 ) ) ;
#38257=AXIS2_PLACEMENT_3D ( 'NONE', #23062, #13321, #42679 ) ;
#38374=LINE ( 'NONE', #28470, #41484 ) ;
#38490=DIRECTION ( 'NONE',  ( -0.000000000000000000, -0.000000000000000000, 1.000000000000000000 ) ) ;
#38513=CARTESIAN_POINT ( 'NONE',  ( 80.00000000000002842, 39.99999999999999289, -160.0000000000000000 ) ) ;
#38796=ORIENTED_EDGE ( 'NONE', *, *, #33231, .F. ) ;
#38849=DIRECTION ( 'NONE',  ( -1.000000000000000000, -0.000000000000000000, -0.000000000000000000 ) ) ;
#38945=( NAMED_UNIT ( * ) PLANE_ANGLE_UNIT ( ) SI_UNIT ( $, .RADIAN. ) );
#38983=CIRCLE ( 'NONE', #37620, 20.00000000000000355 ) ;
#39050=SHAPE_DEFINITION_REPRESENTATION ( #17307, #10057 ) ;
#39176=VECTOR ( 'NONE', #917, 1000.000000000000000 ) ;
#39192=LINE ( 'NONE', #16504, #14810 ) ;
#39258=EDGE_LOOP ( 'NONE', ( #11759, #33145 ) ) ;
#39373=DIRECTION ( 'NONE',  ( 0.000000000000000000, 0.000000000000000000, -1.000000000000000000 ) ) ;
#39387=EDGE_LOOP ( 'NONE', ( #30093, #19355, #22763, #6921 ) ) ;
#39411=FACE_OUTER_BOUND ( 'NONE', #39387, .T. ) ;
#39526=DIRECTION ( 'NONE',  ( -0.000000000000000000, -0.000000000000000000, 1.000000000000000000 ) ) ;
#39539=CARTESIAN_POINT ( 'NONE',  ( 80.00000000000002842, 19.99999999999999289, -170.0000000000000000 ) ) ;
#39678=ORIENTED_EDGE ( 'NONE', *, *, #28973, .T. ) ;
#39784=UNCERTAINTY_MEASURE_WITH_UNIT (LENGTH_MEASURE( 1.000000000000000082E-05 ), #40886, 'distance_accuracy_value', 'NONE');
#39793=CARTESIAN_POINT ( 'NONE',  ( -79.99999999999992895, 19.99999999999998934, -170.0000000000000000 ) ) ;
#39830=LINE ( 'NONE', #6411, #20094 ) ;
#39848=FACE_OUTER_BOUND ( 'NONE', #18772, .T. ) ;
#39910=DIRECTION ( 'NONE',  ( 0.000000000000000000, 0.000000000000000000, -1.000000000000000000 ) ) ;
#39998=AXIS2_PLACEMENT_3D ( 'NONE', #24743, #11112, #37889 ) ;
#40050=EDGE_LOOP ( 'NONE', ( #39678, #36819, #33151, #28820, #41679, #25638, #42484, #27681 ) ) ;
#40227=ORIENTED_EDGE ( 'NONE', *, *, #9361, .T. ) ;
#40566=VERTEX_POINT ( 'NONE', #24312 ) ;
#40722=FACE_BOUND ( 'NONE', #2068, .T. ) ;
#40780=VECTOR ( 'NONE', #21369, 1000.000000000000000 ) ;
#40803=DIRECTION ( 'NONE',  ( -1.000000000000000000, 0.000000000000000000, 0.000000000000000000 ) ) ;
#40833=CIRCLE ( 'NONE', #35360, 25.00000000000000000 ) ;
#40886=( LENGTH_UNIT ( ) NAMED_UNIT ( * ) SI_UNIT ( .MILLI., .METRE. ) );
#40903=DIRECTION ( 'NONE',  ( -1.000000000000000000, 0.000000000000000000, -0.000000000000000000 ) ) ;
#40941=ORIENTED_EDGE ( 'NONE', *, *, #21192, .F. ) ;
#41104=CARTESIAN_POINT ( 'NONE',  ( -99.99999999999994316, -40.00000000000000711, -170.0000000000000000 ) ) ;
#41143=ADVANCED_FACE ( 'NONE', ( #27584, #40722 ), #24572, .T. ) ;
#41145=DIRECTION ( 'NONE',  ( -1.000000000000000000, 0.000000000000000000, -0.000000000000000000 ) ) ;
#41194=EDGE_LOOP ( 'NONE', ( #3812, #17214, #9492, #34130 ) ) ;
#41382=ADVANCED_FACE ( 'NONE', ( #31906 ), #22593, .T. ) ;
#41484=VECTOR ( 'NONE', #8607, 1000.000000000000000 ) ;
#41556=DIRECTION ( 'NONE',  ( 0.000000000000000000, 0.000000000000000000, -1.000000000000000000 ) ) ;
#41679=ORIENTED_EDGE ( 'NONE', *, *, #16436, .T. ) ;
#41740=EDGE_CURVE ( 'NONE', #9407, #27758, #2180, .T. ) ;
#41802=VERTEX_POINT ( 'NONE', #36869 ) ;
#41909=VECTOR ( 'NONE', #41556, 1000.000000000000000 ) ;
#41943=AXIS2_PLACEMENT_3D ( 'NONE', #15595, #38490, #28797 ) ;
#42312=ORIENTED_EDGE ( 'NONE', *, *, #645, .T. ) ;
#42446=DIRECTION ( 'NONE',  ( -1.734723475976807094E-16, -1.000000000000000000, -0.000000000000000000 ) ) ;
#42484=ORIENTED_EDGE ( 'NONE', *, *, #31256, .T. ) ;
#42534=DIRECTION ( 'NONE',  ( -0.000000000000000000, -0.000000000000000000, 1.000000000000000000 ) ) ;
#42679=DIRECTION ( 'NONE',  ( -1.000000000000000000, 0.000000000000000000, 0.000000000000000000 ) ) ;
#42697=COLOUR_RGB('Deep Blue', 0.09019608, 0.27058824, 0.51372549);
#42698=FILL_AREA_STYLE_COLOUR('',#42697);
#42699=FILL_AREA_STYLE('',(#42698));
#42700=SURFACE_STYLE_FILL_AREA(#42699);
#42701=SURFACE_SIDE_STYLE('',(#42700));
#42702=SURFACE_STYLE_USAGE(.BOTH.,#42701);
#42703=PRESENTATION_STYLE_ASSIGNMENT((#42702));
#42743=STYLED_ITEM('',(#42703),#1204);
#42744=MECHANICAL_DESIGN_GEOMETRIC_PRESENTATION_REPRESENTATION('',(#42743),#28334);
ENDSEC;
END-ISO-10303-21;
